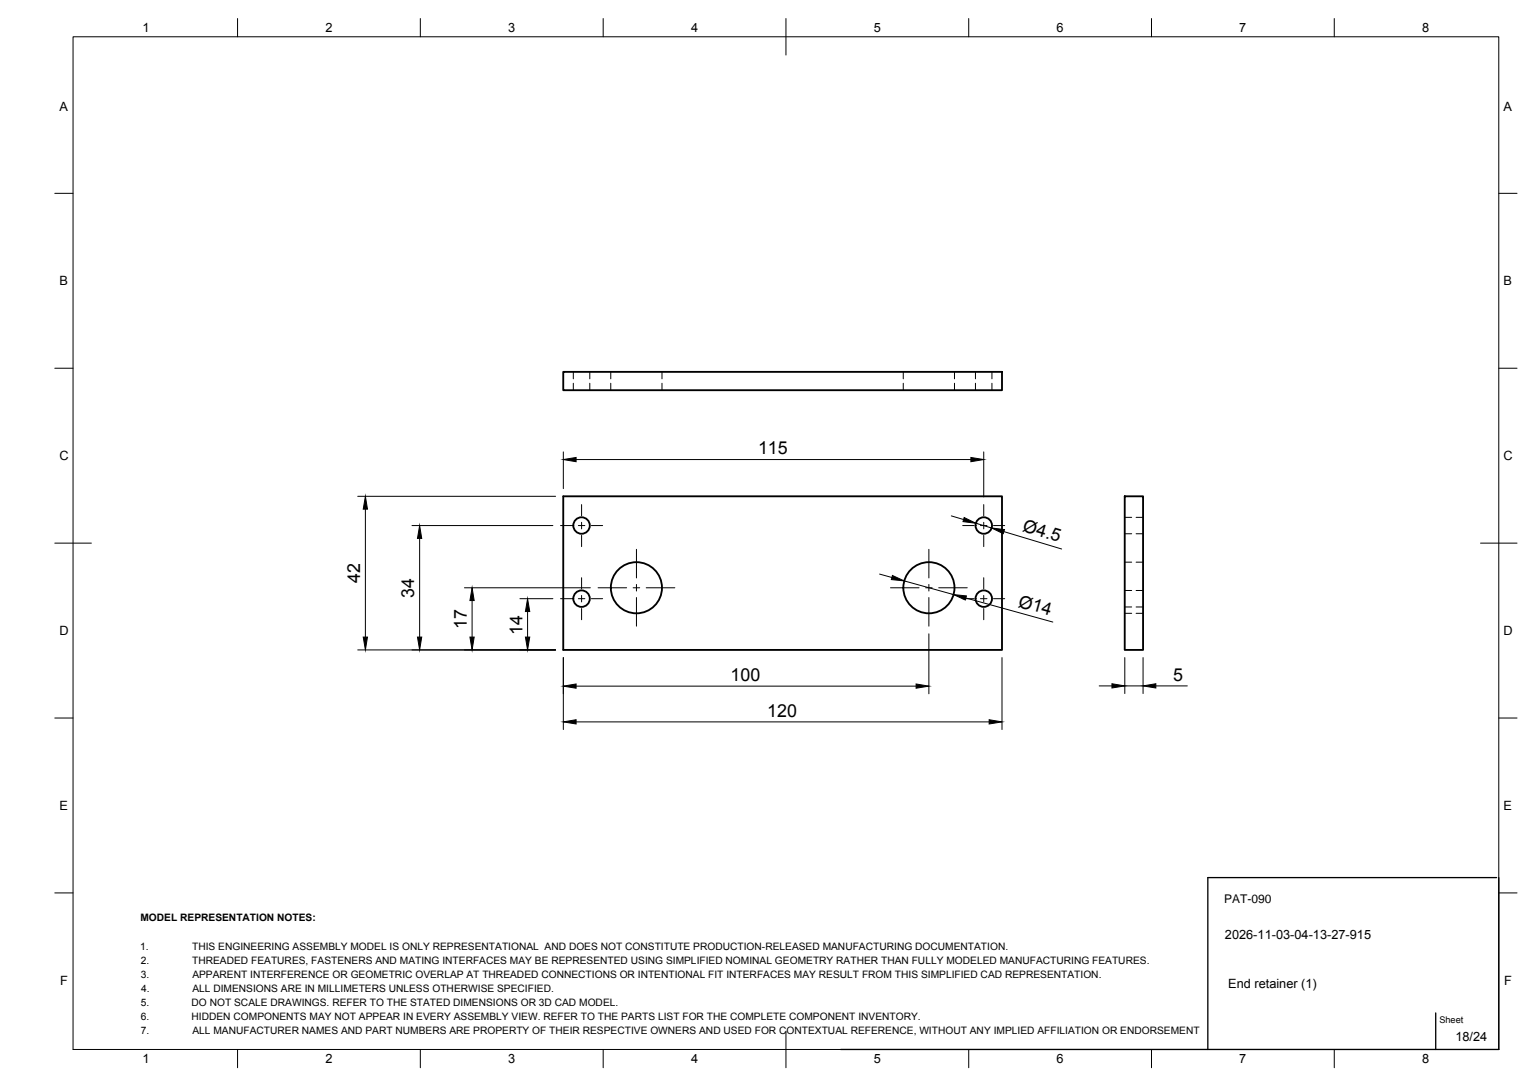
ISO-10303-21;
HEADER;
/* Generated by software containing ST-Developer
 * from STEP Tools, Inc. (www.steptools.com) 
 */

FILE_DESCRIPTION(
/* description */ ('Round-Shaft Linear Stage with Ball Bushings'),
/* implementation_level */ '2;1');

FILE_NAME(
/* name */ 'End retainer (1).step',
/* time_stamp */ '2026-10-27T10:47:55-07:00',
/* author */ (''),
/* organization */ (''),
/* preprocessor_version */ 'ST-DEVELOPER v20.2',
/* originating_system */ 'Autodesk Translation Framework v15.17.0.0',
/* authorisation */ '');

FILE_SCHEMA (('AUTOMOTIVE_DESIGN { 1 0 10303 214 3 1 1 }'));
ENDSEC;

DATA;
#10=MECHANICAL_DESIGN_GEOMETRIC_PRESENTATION_REPRESENTATION('',(#314),#7835);
#272=SHAPE_REPRESENTATION_RELATIONSHIP('SRR','None',#7961,#293);
#293=ADVANCED_BREP_SHAPE_REPRESENTATION('',(#334),#7825);
#314=STYLED_ITEM('',(#8130),#334);
#334=MANIFOLD_SOLID_BREP('Body1',#4405);
#419=FACE_BOUND('',#1110,.T.);
#420=FACE_BOUND('',#1111,.T.);
#421=FACE_BOUND('',#1112,.T.);
#422=FACE_BOUND('',#1113,.T.);
#423=FACE_BOUND('',#1114,.T.);
#424=FACE_BOUND('',#1115,.T.);
#425=FACE_BOUND('',#1118,.T.);
#426=FACE_BOUND('',#1119,.T.);
#427=FACE_BOUND('',#1120,.T.);
#428=FACE_BOUND('',#1121,.T.);
#429=FACE_BOUND('',#1122,.T.);
#430=FACE_BOUND('',#1123,.T.);
#550=PLANE('',#4946);
#551=PLANE('',#4947);
#552=PLANE('',#4948);
#553=PLANE('',#4949);
#554=PLANE('',#4950);
#555=PLANE('',#4951);
#766=FACE_OUTER_BOUND('',#1102,.T.);
#767=FACE_OUTER_BOUND('',#1103,.T.);
#768=FACE_OUTER_BOUND('',#1104,.T.);
#769=FACE_OUTER_BOUND('',#1105,.T.);
#770=FACE_OUTER_BOUND('',#1106,.T.);
#771=FACE_OUTER_BOUND('',#1107,.T.);
#772=FACE_OUTER_BOUND('',#1108,.T.);
#773=FACE_OUTER_BOUND('',#1109,.T.);
#774=FACE_OUTER_BOUND('',#1116,.T.);
#775=FACE_OUTER_BOUND('',#1117,.T.);
#776=FACE_OUTER_BOUND('',#1124,.T.);
#777=FACE_OUTER_BOUND('',#1125,.T.);
#1102=EDGE_LOOP('',(#3626,#3627,#3628,#3629));
#1103=EDGE_LOOP('',(#3630,#3631,#3632,#3633));
#1104=EDGE_LOOP('',(#3634,#3635,#3636,#3637));
#1105=EDGE_LOOP('',(#3638,#3639,#3640,#3641));
#1106=EDGE_LOOP('',(#3642,#3643,#3644,#3645));
#1107=EDGE_LOOP('',(#3646,#3647,#3648,#3649));
#1108=EDGE_LOOP('',(#3650,#3651,#3652,#3653));
#1109=EDGE_LOOP('',(#3654,#3655,#3656,#3657));
#1110=EDGE_LOOP('',(#3658));
#1111=EDGE_LOOP('',(#3659));
#1112=EDGE_LOOP('',(#3660));
#1113=EDGE_LOOP('',(#3661));
#1114=EDGE_LOOP('',(#3662));
#1115=EDGE_LOOP('',(#3663));
#1116=EDGE_LOOP('',(#3664,#3665,#3666,#3667));
#1117=EDGE_LOOP('',(#3668,#3669,#3670,#3671));
#1118=EDGE_LOOP('',(#3672));
#1119=EDGE_LOOP('',(#3673));
#1120=EDGE_LOOP('',(#3674));
#1121=EDGE_LOOP('',(#3675));
#1122=EDGE_LOOP('',(#3676));
#1123=EDGE_LOOP('',(#3677));
#1124=EDGE_LOOP('',(#3678,#3679,#3680,#3681));
#1125=EDGE_LOOP('',(#3682,#3683,#3684,#3685));
#1452=LINE('',#7265,#1792);
#1453=LINE('',#7271,#1793);
#1454=LINE('',#7277,#1794);
#1455=LINE('',#7283,#1795);
#1456=LINE('',#7289,#1796);
#1457=LINE('',#7295,#1797);
#1458=LINE('',#7300,#1798);
#1459=LINE('',#7302,#1799);
#1460=LINE('',#7304,#1800);
#1461=LINE('',#7305,#1801);
#1462=LINE('',#7308,#1802);
#1463=LINE('',#7310,#1803);
#1464=LINE('',#7311,#1804);
#1465=LINE('',#7314,#1805);
#1466=LINE('',#7316,#1806);
#1467=LINE('',#7317,#1807);
#1468=LINE('',#7319,#1808);
#1469=LINE('',#7320,#1809);
#1792=VECTOR('',#5941,0.225);
#1793=VECTOR('',#5948,0.225);
#1794=VECTOR('',#5955,0.225);
#1795=VECTOR('',#5962,0.225);
#1796=VECTOR('',#5969,0.7);
#1797=VECTOR('',#5976,0.7);
#1798=VECTOR('',#5981,1.);
#1799=VECTOR('',#5982,1.);
#1800=VECTOR('',#5983,1.);
#1801=VECTOR('',#5984,1.);
#1802=VECTOR('',#5987,1.);
#1803=VECTOR('',#5988,1.);
#1804=VECTOR('',#5989,1.);
#1805=VECTOR('',#5992,1.);
#1806=VECTOR('',#5993,1.);
#1807=VECTOR('',#5994,1.);
#1808=VECTOR('',#5997,1.);
#1809=VECTOR('',#5998,1.);
#2042=CIRCLE('',#4929,0.225);
#2043=CIRCLE('',#4930,0.225);
#2044=CIRCLE('',#4932,0.225);
#2045=CIRCLE('',#4933,0.225);
#2046=CIRCLE('',#4935,0.225);
#2047=CIRCLE('',#4936,0.225);
#2048=CIRCLE('',#4938,0.225);
#2049=CIRCLE('',#4939,0.225);
#2050=CIRCLE('',#4941,0.7);
#2051=CIRCLE('',#4942,0.7);
#2052=CIRCLE('',#4944,0.7);
#2053=CIRCLE('',#4945,0.7);
#2327=VERTEX_POINT('',#7262);
#2328=VERTEX_POINT('',#7264);
#2329=VERTEX_POINT('',#7268);
#2330=VERTEX_POINT('',#7270);
#2331=VERTEX_POINT('',#7274);
#2332=VERTEX_POINT('',#7276);
#2333=VERTEX_POINT('',#7280);
#2334=VERTEX_POINT('',#7282);
#2335=VERTEX_POINT('',#7286);
#2336=VERTEX_POINT('',#7288);
#2337=VERTEX_POINT('',#7292);
#2338=VERTEX_POINT('',#7294);
#2339=VERTEX_POINT('',#7298);
#2340=VERTEX_POINT('',#7299);
#2341=VERTEX_POINT('',#7301);
#2342=VERTEX_POINT('',#7303);
#2343=VERTEX_POINT('',#7307);
#2344=VERTEX_POINT('',#7309);
#2345=VERTEX_POINT('',#7313);
#2346=VERTEX_POINT('',#7315);
#2781=EDGE_CURVE('',#2327,#2327,#2042,.T.);
#2782=EDGE_CURVE('',#2327,#2328,#1452,.T.);
#2783=EDGE_CURVE('',#2328,#2328,#2043,.T.);
#2784=EDGE_CURVE('',#2329,#2329,#2044,.T.);
#2785=EDGE_CURVE('',#2329,#2330,#1453,.T.);
#2786=EDGE_CURVE('',#2330,#2330,#2045,.T.);
#2787=EDGE_CURVE('',#2331,#2331,#2046,.T.);
#2788=EDGE_CURVE('',#2331,#2332,#1454,.T.);
#2789=EDGE_CURVE('',#2332,#2332,#2047,.T.);
#2790=EDGE_CURVE('',#2333,#2333,#2048,.T.);
#2791=EDGE_CURVE('',#2333,#2334,#1455,.T.);
#2792=EDGE_CURVE('',#2334,#2334,#2049,.T.);
#2793=EDGE_CURVE('',#2335,#2335,#2050,.T.);
#2794=EDGE_CURVE('',#2335,#2336,#1456,.T.);
#2795=EDGE_CURVE('',#2336,#2336,#2051,.T.);
#2796=EDGE_CURVE('',#2337,#2337,#2052,.T.);
#2797=EDGE_CURVE('',#2337,#2338,#1457,.T.);
#2798=EDGE_CURVE('',#2338,#2338,#2053,.T.);
#2799=EDGE_CURVE('',#2339,#2340,#1458,.T.);
#2800=EDGE_CURVE('',#2340,#2341,#1459,.T.);
#2801=EDGE_CURVE('',#2342,#2341,#1460,.T.);
#2802=EDGE_CURVE('',#2339,#2342,#1461,.T.);
#2803=EDGE_CURVE('',#2343,#2339,#1462,.T.);
#2804=EDGE_CURVE('',#2344,#2342,#1463,.T.);
#2805=EDGE_CURVE('',#2343,#2344,#1464,.T.);
#2806=EDGE_CURVE('',#2345,#2343,#1465,.T.);
#2807=EDGE_CURVE('',#2346,#2344,#1466,.T.);
#2808=EDGE_CURVE('',#2345,#2346,#1467,.T.);
#2809=EDGE_CURVE('',#2340,#2345,#1468,.T.);
#2810=EDGE_CURVE('',#2341,#2346,#1469,.T.);
#3626=ORIENTED_EDGE('',*,*,#2781,.F.);
#3627=ORIENTED_EDGE('',*,*,#2782,.T.);
#3628=ORIENTED_EDGE('',*,*,#2783,.F.);
#3629=ORIENTED_EDGE('',*,*,#2782,.F.);
#3630=ORIENTED_EDGE('',*,*,#2784,.F.);
#3631=ORIENTED_EDGE('',*,*,#2785,.T.);
#3632=ORIENTED_EDGE('',*,*,#2786,.F.);
#3633=ORIENTED_EDGE('',*,*,#2785,.F.);
#3634=ORIENTED_EDGE('',*,*,#2787,.F.);
#3635=ORIENTED_EDGE('',*,*,#2788,.T.);
#3636=ORIENTED_EDGE('',*,*,#2789,.F.);
#3637=ORIENTED_EDGE('',*,*,#2788,.F.);
#3638=ORIENTED_EDGE('',*,*,#2790,.F.);
#3639=ORIENTED_EDGE('',*,*,#2791,.T.);
#3640=ORIENTED_EDGE('',*,*,#2792,.F.);
#3641=ORIENTED_EDGE('',*,*,#2791,.F.);
#3642=ORIENTED_EDGE('',*,*,#2793,.F.);
#3643=ORIENTED_EDGE('',*,*,#2794,.T.);
#3644=ORIENTED_EDGE('',*,*,#2795,.F.);
#3645=ORIENTED_EDGE('',*,*,#2794,.F.);
#3646=ORIENTED_EDGE('',*,*,#2796,.F.);
#3647=ORIENTED_EDGE('',*,*,#2797,.T.);
#3648=ORIENTED_EDGE('',*,*,#2798,.F.);
#3649=ORIENTED_EDGE('',*,*,#2797,.F.);
#3650=ORIENTED_EDGE('',*,*,#2799,.T.);
#3651=ORIENTED_EDGE('',*,*,#2800,.T.);
#3652=ORIENTED_EDGE('',*,*,#2801,.F.);
#3653=ORIENTED_EDGE('',*,*,#2802,.F.);
#3654=ORIENTED_EDGE('',*,*,#2803,.T.);
#3655=ORIENTED_EDGE('',*,*,#2802,.T.);
#3656=ORIENTED_EDGE('',*,*,#2804,.F.);
#3657=ORIENTED_EDGE('',*,*,#2805,.F.);
#3658=ORIENTED_EDGE('',*,*,#2798,.T.);
#3659=ORIENTED_EDGE('',*,*,#2795,.T.);
#3660=ORIENTED_EDGE('',*,*,#2792,.T.);
#3661=ORIENTED_EDGE('',*,*,#2789,.T.);
#3662=ORIENTED_EDGE('',*,*,#2786,.T.);
#3663=ORIENTED_EDGE('',*,*,#2783,.T.);
#3664=ORIENTED_EDGE('',*,*,#2806,.T.);
#3665=ORIENTED_EDGE('',*,*,#2805,.T.);
#3666=ORIENTED_EDGE('',*,*,#2807,.F.);
#3667=ORIENTED_EDGE('',*,*,#2808,.F.);
#3668=ORIENTED_EDGE('',*,*,#2809,.T.);
#3669=ORIENTED_EDGE('',*,*,#2808,.T.);
#3670=ORIENTED_EDGE('',*,*,#2810,.F.);
#3671=ORIENTED_EDGE('',*,*,#2800,.F.);
#3672=ORIENTED_EDGE('',*,*,#2796,.T.);
#3673=ORIENTED_EDGE('',*,*,#2793,.T.);
#3674=ORIENTED_EDGE('',*,*,#2790,.T.);
#3675=ORIENTED_EDGE('',*,*,#2787,.T.);
#3676=ORIENTED_EDGE('',*,*,#2784,.T.);
#3677=ORIENTED_EDGE('',*,*,#2781,.T.);
#3678=ORIENTED_EDGE('',*,*,#2810,.T.);
#3679=ORIENTED_EDGE('',*,*,#2807,.T.);
#3680=ORIENTED_EDGE('',*,*,#2804,.T.);
#3681=ORIENTED_EDGE('',*,*,#2801,.T.);
#3682=ORIENTED_EDGE('',*,*,#2809,.F.);
#3683=ORIENTED_EDGE('',*,*,#2799,.F.);
#3684=ORIENTED_EDGE('',*,*,#2803,.F.);
#3685=ORIENTED_EDGE('',*,*,#2806,.F.);
#4106=CYLINDRICAL_SURFACE('',#4928,0.225);
#4107=CYLINDRICAL_SURFACE('',#4931,0.225);
#4108=CYLINDRICAL_SURFACE('',#4934,0.225);
#4109=CYLINDRICAL_SURFACE('',#4937,0.225);
#4110=CYLINDRICAL_SURFACE('',#4940,0.7);
#4111=CYLINDRICAL_SURFACE('',#4943,0.7);
#4285=ADVANCED_FACE('',(#766),#4106,.F.);
#4286=ADVANCED_FACE('',(#767),#4107,.F.);
#4287=ADVANCED_FACE('',(#768),#4108,.F.);
#4288=ADVANCED_FACE('',(#769),#4109,.F.);
#4289=ADVANCED_FACE('',(#770),#4110,.F.);
#4290=ADVANCED_FACE('',(#771),#4111,.F.);
#4291=ADVANCED_FACE('',(#772),#550,.T.);
#4292=ADVANCED_FACE('',(#773,#419,#420,#421,#422,#423,#424),#551,.T.);
#4293=ADVANCED_FACE('',(#774),#552,.T.);
#4294=ADVANCED_FACE('',(#775,#425,#426,#427,#428,#429,#430),#553,.T.);
#4295=ADVANCED_FACE('',(#776),#554,.T.);
#4296=ADVANCED_FACE('',(#777),#555,.F.);
#4405=CLOSED_SHELL('',(#4285,#4286,#4287,#4288,#4289,#4290,#4291,#4292,
#4293,#4294,#4295,#4296));
#4927=AXIS2_PLACEMENT_3D('',#7260,#5935,#5936);
#4928=AXIS2_PLACEMENT_3D('',#7261,#5937,#5938);
#4929=AXIS2_PLACEMENT_3D('',#7263,#5939,#5940);
#4930=AXIS2_PLACEMENT_3D('',#7266,#5942,#5943);
#4931=AXIS2_PLACEMENT_3D('',#7267,#5944,#5945);
#4932=AXIS2_PLACEMENT_3D('',#7269,#5946,#5947);
#4933=AXIS2_PLACEMENT_3D('',#7272,#5949,#5950);
#4934=AXIS2_PLACEMENT_3D('',#7273,#5951,#5952);
#4935=AXIS2_PLACEMENT_3D('',#7275,#5953,#5954);
#4936=AXIS2_PLACEMENT_3D('',#7278,#5956,#5957);
#4937=AXIS2_PLACEMENT_3D('',#7279,#5958,#5959);
#4938=AXIS2_PLACEMENT_3D('',#7281,#5960,#5961);
#4939=AXIS2_PLACEMENT_3D('',#7284,#5963,#5964);
#4940=AXIS2_PLACEMENT_3D('',#7285,#5965,#5966);
#4941=AXIS2_PLACEMENT_3D('',#7287,#5967,#5968);
#4942=AXIS2_PLACEMENT_3D('',#7290,#5970,#5971);
#4943=AXIS2_PLACEMENT_3D('',#7291,#5972,#5973);
#4944=AXIS2_PLACEMENT_3D('',#7293,#5974,#5975);
#4945=AXIS2_PLACEMENT_3D('',#7296,#5977,#5978);
#4946=AXIS2_PLACEMENT_3D('',#7297,#5979,#5980);
#4947=AXIS2_PLACEMENT_3D('',#7306,#5985,#5986);
#4948=AXIS2_PLACEMENT_3D('',#7312,#5990,#5991);
#4949=AXIS2_PLACEMENT_3D('',#7318,#5995,#5996);
#4950=AXIS2_PLACEMENT_3D('',#7321,#5999,#6000);
#4951=AXIS2_PLACEMENT_3D('',#7322,#6001,#6002);
#5935=DIRECTION('axis',(0.,0.,1.));
#5936=DIRECTION('refdir',(1.,0.,0.));
#5937=DIRECTION('center_axis',(1.,0.,0.));
#5938=DIRECTION('ref_axis',(0.,0.,-1.));
#5939=DIRECTION('center_axis',(1.,0.,0.));
#5940=DIRECTION('ref_axis',(0.,0.,-1.));
#5941=DIRECTION('',(1.,0.,0.));
#5942=DIRECTION('center_axis',(-1.,0.,0.));
#5943=DIRECTION('ref_axis',(0.,0.,-1.));
#5944=DIRECTION('center_axis',(1.,0.,0.));
#5945=DIRECTION('ref_axis',(0.,0.,-1.));
#5946=DIRECTION('center_axis',(1.,0.,0.));
#5947=DIRECTION('ref_axis',(0.,0.,-1.));
#5948=DIRECTION('',(1.,0.,0.));
#5949=DIRECTION('center_axis',(-1.,0.,0.));
#5950=DIRECTION('ref_axis',(0.,0.,-1.));
#5951=DIRECTION('center_axis',(1.,0.,0.));
#5952=DIRECTION('ref_axis',(0.,0.,-1.));
#5953=DIRECTION('center_axis',(1.,0.,0.));
#5954=DIRECTION('ref_axis',(0.,0.,-1.));
#5955=DIRECTION('',(1.,0.,0.));
#5956=DIRECTION('center_axis',(-1.,0.,0.));
#5957=DIRECTION('ref_axis',(0.,0.,-1.));
#5958=DIRECTION('center_axis',(1.,0.,0.));
#5959=DIRECTION('ref_axis',(0.,0.,-1.));
#5960=DIRECTION('center_axis',(1.,0.,0.));
#5961=DIRECTION('ref_axis',(0.,0.,-1.));
#5962=DIRECTION('',(1.,0.,0.));
#5963=DIRECTION('center_axis',(-1.,0.,0.));
#5964=DIRECTION('ref_axis',(0.,0.,-1.));
#5965=DIRECTION('center_axis',(1.,0.,0.));
#5966=DIRECTION('ref_axis',(0.,0.,-1.));
#5967=DIRECTION('center_axis',(1.,0.,0.));
#5968=DIRECTION('ref_axis',(0.,0.,-1.));
#5969=DIRECTION('',(1.,0.,0.));
#5970=DIRECTION('center_axis',(-1.,0.,0.));
#5971=DIRECTION('ref_axis',(0.,0.,-1.));
#5972=DIRECTION('center_axis',(1.,0.,0.));
#5973=DIRECTION('ref_axis',(0.,0.,-1.));
#5974=DIRECTION('center_axis',(1.,0.,0.));
#5975=DIRECTION('ref_axis',(0.,0.,-1.));
#5976=DIRECTION('',(1.,0.,0.));
#5977=DIRECTION('center_axis',(-1.,0.,0.));
#5978=DIRECTION('ref_axis',(0.,0.,-1.));
#5979=DIRECTION('center_axis',(0.,1.,0.));
#5980=DIRECTION('ref_axis',(-1.,0.,0.));
#5981=DIRECTION('',(-1.,0.,0.));
#5982=DIRECTION('',(0.,0.,1.));
#5983=DIRECTION('',(-1.,0.,0.));
#5984=DIRECTION('',(0.,0.,1.));
#5985=DIRECTION('center_axis',(1.,0.,0.));
#5986=DIRECTION('ref_axis',(0.,1.,0.));
#5987=DIRECTION('',(0.,1.,0.));
#5988=DIRECTION('',(0.,1.,0.));
#5989=DIRECTION('',(0.,0.,1.));
#5990=DIRECTION('center_axis',(0.,-1.,0.));
#5991=DIRECTION('ref_axis',(1.,0.,0.));
#5992=DIRECTION('',(1.,0.,0.));
#5993=DIRECTION('',(1.,0.,0.));
#5994=DIRECTION('',(0.,0.,1.));
#5995=DIRECTION('center_axis',(-1.,0.,0.));
#5996=DIRECTION('ref_axis',(0.,-1.,0.));
#5997=DIRECTION('',(0.,-1.,0.));
#5998=DIRECTION('',(0.,-1.,0.));
#5999=DIRECTION('center_axis',(0.,0.,1.));
#6000=DIRECTION('ref_axis',(1.,0.,0.));
#6001=DIRECTION('center_axis',(0.,0.,1.));
#6002=DIRECTION('ref_axis',(1.,0.,0.));
#7260=CARTESIAN_POINT('',(0.,0.,0.));
#7261=CARTESIAN_POINT('Origin',(19.4,5.5,3.));
#7262=CARTESIAN_POINT('',(19.5,5.5,3.225));
#7263=CARTESIAN_POINT('Origin',(19.5,5.5,3.));
#7264=CARTESIAN_POINT('',(20.,5.5,3.225));
#7265=CARTESIAN_POINT('',(19.4,5.5,3.225));
#7266=CARTESIAN_POINT('Origin',(20.,5.5,3.));
#7267=CARTESIAN_POINT('Origin',(19.4,-5.5,5.));
#7268=CARTESIAN_POINT('',(19.5,-5.5,5.225));
#7269=CARTESIAN_POINT('Origin',(19.5,-5.5,5.));
#7270=CARTESIAN_POINT('',(20.,-5.5,5.225));
#7271=CARTESIAN_POINT('',(19.4,-5.5,5.225));
#7272=CARTESIAN_POINT('Origin',(20.,-5.5,5.));
#7273=CARTESIAN_POINT('Origin',(19.4,-5.5,3.));
#7274=CARTESIAN_POINT('',(19.5,-5.5,3.225));
#7275=CARTESIAN_POINT('Origin',(19.5,-5.5,3.));
#7276=CARTESIAN_POINT('',(20.,-5.5,3.225));
#7277=CARTESIAN_POINT('',(19.4,-5.5,3.225));
#7278=CARTESIAN_POINT('Origin',(20.,-5.5,3.));
#7279=CARTESIAN_POINT('Origin',(19.4,5.5,5.));
#7280=CARTESIAN_POINT('',(19.5,5.5,5.225));
#7281=CARTESIAN_POINT('Origin',(19.5,5.5,5.));
#7282=CARTESIAN_POINT('',(20.,5.5,5.225));
#7283=CARTESIAN_POINT('',(19.4,5.5,5.225));
#7284=CARTESIAN_POINT('Origin',(20.,5.5,5.));
#7285=CARTESIAN_POINT('Origin',(19.4,-4.,3.3));
#7286=CARTESIAN_POINT('',(19.5,-4.,4.));
#7287=CARTESIAN_POINT('Origin',(19.5,-4.,3.3));
#7288=CARTESIAN_POINT('',(20.,-4.,4.));
#7289=CARTESIAN_POINT('',(19.4,-4.,4.));
#7290=CARTESIAN_POINT('Origin',(20.,-4.,3.3));
#7291=CARTESIAN_POINT('Origin',(19.4,4.,3.3));
#7292=CARTESIAN_POINT('',(19.5,4.,4.));
#7293=CARTESIAN_POINT('Origin',(19.5,4.,3.3));
#7294=CARTESIAN_POINT('',(20.,4.,4.));
#7295=CARTESIAN_POINT('',(19.4,4.,4.));
#7296=CARTESIAN_POINT('Origin',(20.,4.,3.3));
#7297=CARTESIAN_POINT('Origin',(20.,6.,1.6));
#7298=CARTESIAN_POINT('',(20.,6.,1.6));
#7299=CARTESIAN_POINT('',(19.5,6.,1.6));
#7300=CARTESIAN_POINT('',(20.,6.,1.6));
#7301=CARTESIAN_POINT('',(19.5,6.,5.8));
#7302=CARTESIAN_POINT('',(19.5,6.,1.6));
#7303=CARTESIAN_POINT('',(20.,6.,5.8));
#7304=CARTESIAN_POINT('',(20.,6.,5.8));
#7305=CARTESIAN_POINT('',(20.,6.,1.6));
#7306=CARTESIAN_POINT('Origin',(20.,-6.,1.6));
#7307=CARTESIAN_POINT('',(20.,-6.,1.6));
#7308=CARTESIAN_POINT('',(20.,-6.,1.6));
#7309=CARTESIAN_POINT('',(20.,-6.,5.8));
#7310=CARTESIAN_POINT('',(20.,-6.,5.8));
#7311=CARTESIAN_POINT('',(20.,-6.,1.6));
#7312=CARTESIAN_POINT('Origin',(19.5,-6.,1.6));
#7313=CARTESIAN_POINT('',(19.5,-6.,1.6));
#7314=CARTESIAN_POINT('',(19.5,-6.,1.6));
#7315=CARTESIAN_POINT('',(19.5,-6.,5.8));
#7316=CARTESIAN_POINT('',(19.5,-6.,5.8));
#7317=CARTESIAN_POINT('',(19.5,-6.,1.6));
#7318=CARTESIAN_POINT('Origin',(19.5,6.,1.6));
#7319=CARTESIAN_POINT('',(19.5,6.,1.6));
#7320=CARTESIAN_POINT('',(19.5,6.,5.8));
#7321=CARTESIAN_POINT('Origin',(19.75,0.,5.8));
#7322=CARTESIAN_POINT('Origin',(19.75,0.,1.6));
#7799=UNCERTAINTY_MEASURE_WITH_UNIT(LENGTH_MEASURE(0.001),#7836,
'DISTANCE_ACCURACY_VALUE',
'Maximum model space distance between geometric entities at asserted c
onnectivities');
#7809=UNCERTAINTY_MEASURE_WITH_UNIT(LENGTH_MEASURE(0.001),#7836,
'DISTANCE_ACCURACY_VALUE',
'Maximum model space distance between geometric entities at asserted c
onnectivities');
#7825=(
GEOMETRIC_REPRESENTATION_CONTEXT(3)
GLOBAL_UNCERTAINTY_ASSIGNED_CONTEXT((#7799))
GLOBAL_UNIT_ASSIGNED_CONTEXT((#7836,#7838,#7839))
REPRESENTATION_CONTEXT('','3D')
);
#7835=(
GEOMETRIC_REPRESENTATION_CONTEXT(3)
GLOBAL_UNCERTAINTY_ASSIGNED_CONTEXT((#7809))
GLOBAL_UNIT_ASSIGNED_CONTEXT((#7836,#7838,#7839))
REPRESENTATION_CONTEXT('','3D')
);
#7836=(
LENGTH_UNIT()
NAMED_UNIT(*)
SI_UNIT(.CENTI.,.METRE.)
);
#7838=(
NAMED_UNIT(*)
PLANE_ANGLE_UNIT()
SI_UNIT($,.RADIAN.)
);
#7839=(
NAMED_UNIT(*)
SI_UNIT($,.STERADIAN.)
SOLID_ANGLE_UNIT()
);
#7855=SHAPE_DEFINITION_REPRESENTATION(#7880,#7961);
#7880=PRODUCT_DEFINITION_SHAPE('',$,#7987);
#7961=SHAPE_REPRESENTATION('',(#4927),#7825);
#7971=PRODUCT_DEFINITION_CONTEXT('part definition',#8048,'design');
#7987=PRODUCT_DEFINITION('End retainer (1)','End retainer (1)',#8012,#7971);
#8012=PRODUCT_DEFINITION_FORMATION('',$,#8065);
#8048=APPLICATION_CONTEXT(
'Core Data for Automotive Mechanical Design Process');
#8049=PRODUCT_CONTEXT('part definition',#8048,'mechanical');
#8065=PRODUCT('End retainer (1)','End retainer (1)','End retainer (1)',(#8049));
#8124=COLOUR_RGB('Light Blue',0.38,0.62,0.78);
#8125=FILL_AREA_STYLE_COLOUR('',#8124);
#8126=FILL_AREA_STYLE('',(#8125));
#8127=SURFACE_STYLE_FILL_AREA(#8126);
#8128=SURFACE_SIDE_STYLE('',(#8127));
#8129=SURFACE_STYLE_USAGE(.BOTH.,#8128);
#8130=PRESENTATION_STYLE_ASSIGNMENT((#8129));
ENDSEC;
END-ISO-10303-21;
